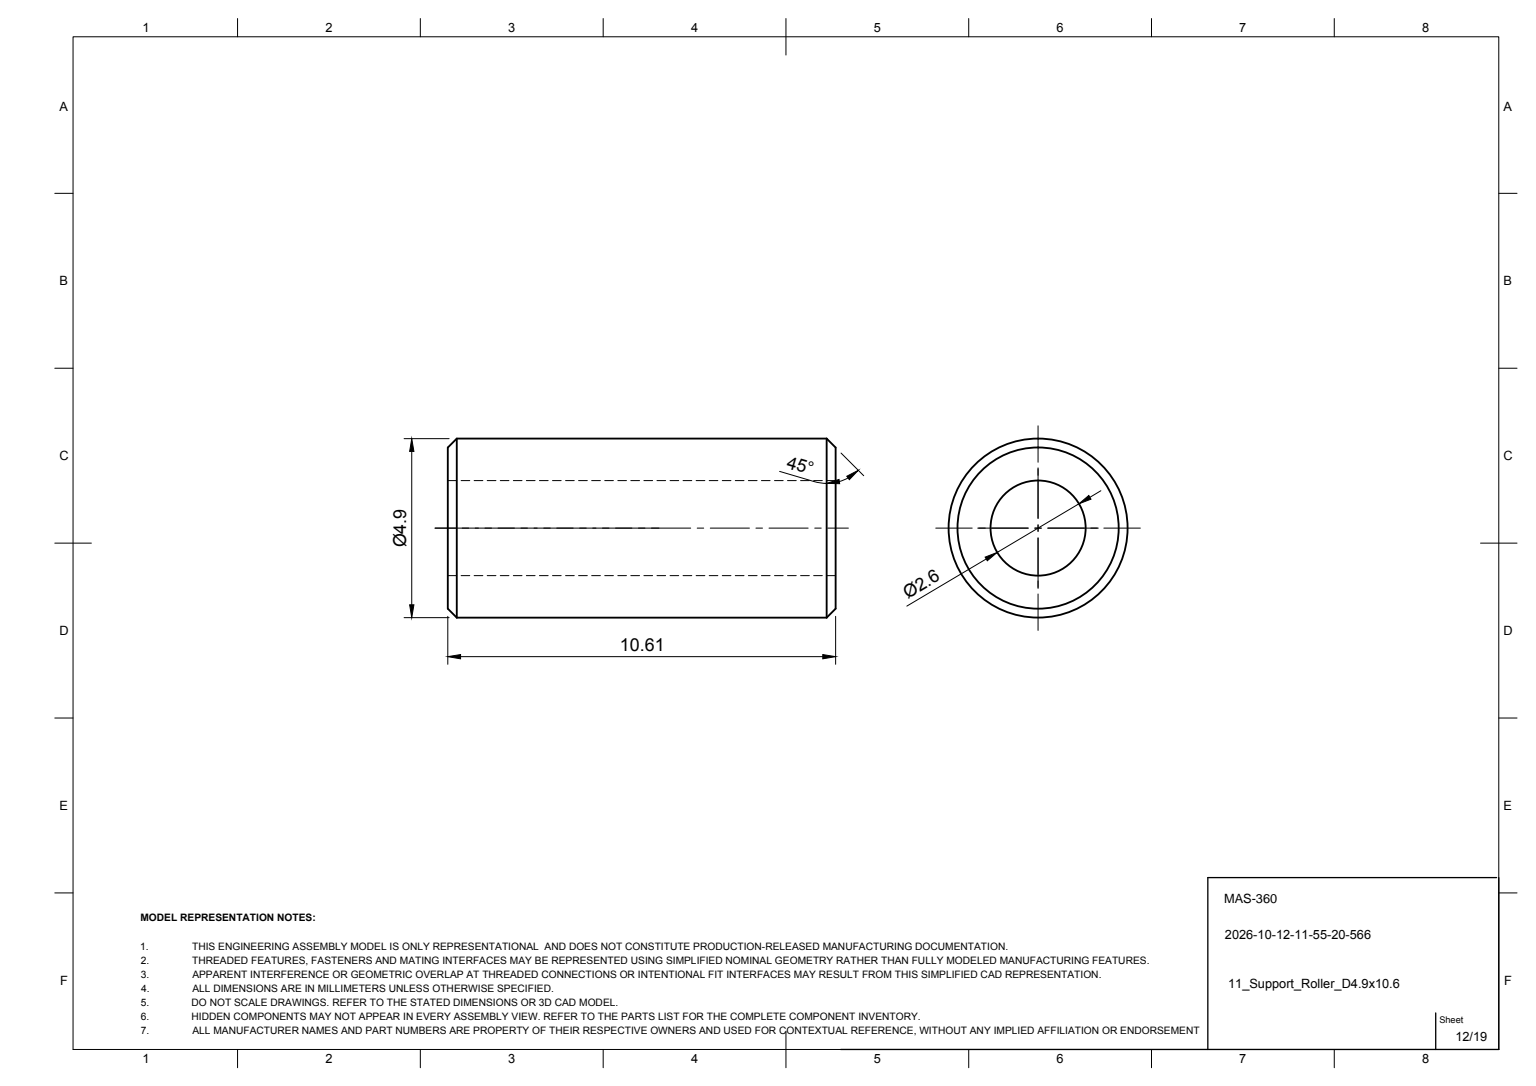
ISO-10303-21;
HEADER;
/* Generated by software containing ST-Developer
 * from STEP Tools, Inc. (www.steptools.com) 
 */

FILE_DESCRIPTION(
/* description */ (''),
/* implementation_level */ '2;1');

FILE_NAME(
/* name */ '11_Support_Roller_D4.9x10.6.step',
/* time_stamp */ '2026-11-04T18:53:29-08:00',
/* author */ (''),
/* organization */ (''),
/* preprocessor_version */ 'ST-DEVELOPER v20.2',
/* originating_system */ 'Autodesk Translation Framework v15.17.0.0',
/* authorisation */ '');

FILE_SCHEMA (('AUTOMOTIVE_DESIGN { 1 0 10303 214 3 1 1 }'));
ENDSEC;

DATA;
#10=MECHANICAL_DESIGN_GEOMETRIC_PRESENTATION_REPRESENTATION('',(#1338),#100031);
#237=CONICAL_SURFACE('',#22405,2.3256,0.785398163397447);
#238=CONICAL_SURFACE('',#22410,2.3256,0.785398163397447);
#1142=CIRCLE('',#22406,2.448);
#1143=CIRCLE('',#22407,2.2032);
#1144=CIRCLE('',#22409,2.448);
#1145=CIRCLE('',#22411,2.2032);
#1146=CIRCLE('',#22413,1.3);
#1147=CIRCLE('',#22415,1.3);
#1302=SHAPE_REPRESENTATION_RELATIONSHIP('SRR','None',#100112,#1320);
#1320=ADVANCED_BREP_SHAPE_REPRESENTATION('',(#1356),#100024);
#1338=STYLED_ITEM('',(#100200),#1356);
#1356=MANIFOLD_SOLID_BREP('Body1',#20128);
#1675=PLANE('',#22412);
#1676=PLANE('',#22416);
#1802=FACE_BOUND('',#7405,.T.);
#1803=FACE_BOUND('',#7408,.T.);
#3241=LINE('',#99809,#4528);
#3242=LINE('',#99814,#4529);
#3243=LINE('',#99817,#4530);
#3244=LINE('',#99825,#4531);
#4528=VECTOR('',#27932,2.3256);
#4529=VECTOR('',#27939,2.448);
#4530=VECTOR('',#27942,2.3256);
#4531=VECTOR('',#27953,1.3);
#5013=CYLINDRICAL_SURFACE('',#22408,2.448);
#5014=CYLINDRICAL_SURFACE('',#22414,1.3);
#6136=FACE_OUTER_BOUND('',#7401,.T.);
#6137=FACE_OUTER_BOUND('',#7402,.T.);
#6138=FACE_OUTER_BOUND('',#7403,.T.);
#6139=FACE_OUTER_BOUND('',#7404,.T.);
#6140=FACE_OUTER_BOUND('',#7406,.T.);
#6141=FACE_OUTER_BOUND('',#7407,.T.);
#7401=EDGE_LOOP('',(#18715,#18716,#18717,#18718));
#7402=EDGE_LOOP('',(#18719,#18720,#18721,#18722));
#7403=EDGE_LOOP('',(#18723,#18724,#18725,#18726));
#7404=EDGE_LOOP('',(#18727));
#7405=EDGE_LOOP('',(#18728));
#7406=EDGE_LOOP('',(#18729,#18730,#18731,#18732));
#7407=EDGE_LOOP('',(#18733));
#7408=EDGE_LOOP('',(#18734));
#9883=VERTEX_POINT('',#99806);
#9884=VERTEX_POINT('',#99808);
#9885=VERTEX_POINT('',#99812);
#9886=VERTEX_POINT('',#99816);
#9887=VERTEX_POINT('',#99820);
#9888=VERTEX_POINT('',#99823);
#12832=EDGE_CURVE('',#9883,#9883,#1142,.T.);
#12833=EDGE_CURVE('',#9883,#9884,#3241,.T.);
#12834=EDGE_CURVE('',#9884,#9884,#1143,.T.);
#12835=EDGE_CURVE('',#9885,#9885,#1144,.T.);
#12836=EDGE_CURVE('',#9885,#9883,#3242,.T.);
#12837=EDGE_CURVE('',#9885,#9886,#3243,.T.);
#12838=EDGE_CURVE('',#9886,#9886,#1145,.T.);
#12839=EDGE_CURVE('',#9887,#9887,#1146,.T.);
#12840=EDGE_CURVE('',#9888,#9888,#1147,.T.);
#12841=EDGE_CURVE('',#9888,#9887,#3244,.T.);
#18715=ORIENTED_EDGE('',*,*,#12832,.F.);
#18716=ORIENTED_EDGE('',*,*,#12833,.T.);
#18717=ORIENTED_EDGE('',*,*,#12834,.T.);
#18718=ORIENTED_EDGE('',*,*,#12833,.F.);
#18719=ORIENTED_EDGE('',*,*,#12835,.F.);
#18720=ORIENTED_EDGE('',*,*,#12836,.T.);
#18721=ORIENTED_EDGE('',*,*,#12832,.T.);
#18722=ORIENTED_EDGE('',*,*,#12836,.F.);
#18723=ORIENTED_EDGE('',*,*,#12835,.T.);
#18724=ORIENTED_EDGE('',*,*,#12837,.T.);
#18725=ORIENTED_EDGE('',*,*,#12838,.F.);
#18726=ORIENTED_EDGE('',*,*,#12837,.F.);
#18727=ORIENTED_EDGE('',*,*,#12838,.T.);
#18728=ORIENTED_EDGE('',*,*,#12839,.F.);
#18729=ORIENTED_EDGE('',*,*,#12840,.F.);
#18730=ORIENTED_EDGE('',*,*,#12841,.T.);
#18731=ORIENTED_EDGE('',*,*,#12839,.T.);
#18732=ORIENTED_EDGE('',*,*,#12841,.F.);
#18733=ORIENTED_EDGE('',*,*,#12834,.F.);
#18734=ORIENTED_EDGE('',*,*,#12840,.T.);
#20070=ADVANCED_FACE('',(#6136),#237,.T.);
#20071=ADVANCED_FACE('',(#6137),#5013,.T.);
#20072=ADVANCED_FACE('',(#6138),#238,.T.);
#20073=ADVANCED_FACE('',(#6139,#1802),#1675,.T.);
#20074=ADVANCED_FACE('',(#6140),#5014,.F.);
#20075=ADVANCED_FACE('',(#6141,#1803),#1676,.T.);
#20128=CLOSED_SHELL('',(#20070,#20071,#20072,#20073,#20074,#20075));
#22404=AXIS2_PLACEMENT_3D('',#99804,#27926,#27927);
#22405=AXIS2_PLACEMENT_3D('',#99805,#27928,#27929);
#22406=AXIS2_PLACEMENT_3D('',#99807,#27930,#27931);
#22407=AXIS2_PLACEMENT_3D('',#99810,#27933,#27934);
#22408=AXIS2_PLACEMENT_3D('',#99811,#27935,#27936);
#22409=AXIS2_PLACEMENT_3D('',#99813,#27937,#27938);
#22410=AXIS2_PLACEMENT_3D('',#99815,#27940,#27941);
#22411=AXIS2_PLACEMENT_3D('',#99818,#27943,#27944);
#22412=AXIS2_PLACEMENT_3D('',#99819,#27945,#27946);
#22413=AXIS2_PLACEMENT_3D('',#99821,#27947,#27948);
#22414=AXIS2_PLACEMENT_3D('',#99822,#27949,#27950);
#22415=AXIS2_PLACEMENT_3D('',#99824,#27951,#27952);
#22416=AXIS2_PLACEMENT_3D('',#99826,#27954,#27955);
#27926=DIRECTION('axis',(0.,0.,1.));
#27927=DIRECTION('refdir',(1.,0.,0.));
#27928=DIRECTION('center_axis',(1.,0.,0.));
#27929=DIRECTION('ref_axis',(0.,1.,0.));
#27930=DIRECTION('center_axis',(1.,0.,0.));
#27931=DIRECTION('ref_axis',(0.,0.,-1.));
#27932=DIRECTION('',(-0.707106781186548,0.707106781186547,8.65956056235492E-17));
#27933=DIRECTION('center_axis',(1.,0.,0.));
#27934=DIRECTION('ref_axis',(0.,0.,-1.));
#27935=DIRECTION('center_axis',(1.,0.,0.));
#27936=DIRECTION('ref_axis',(0.,1.,0.));
#27937=DIRECTION('center_axis',(1.,0.,0.));
#27938=DIRECTION('ref_axis',(0.,0.,-1.));
#27939=DIRECTION('',(-1.,0.,0.));
#27940=DIRECTION('center_axis',(-1.,0.,0.));
#27941=DIRECTION('ref_axis',(0.,1.,0.));
#27942=DIRECTION('',(0.707106781186548,0.707106781186547,-8.65956056235492E-17));
#27943=DIRECTION('center_axis',(1.,0.,0.));
#27944=DIRECTION('ref_axis',(0.,0.,-1.));
#27945=DIRECTION('center_axis',(1.,0.,0.));
#27946=DIRECTION('ref_axis',(0.,0.,-1.));
#27947=DIRECTION('center_axis',(1.,0.,0.));
#27948=DIRECTION('ref_axis',(0.,0.,-1.));
#27949=DIRECTION('center_axis',(1.,0.,0.));
#27950=DIRECTION('ref_axis',(0.,1.,0.));
#27951=DIRECTION('center_axis',(1.,0.,0.));
#27952=DIRECTION('ref_axis',(0.,0.,-1.));
#27953=DIRECTION('',(1.,0.,0.));
#27954=DIRECTION('center_axis',(-1.,0.,0.));
#27955=DIRECTION('ref_axis',(0.,0.,1.));
#99804=CARTESIAN_POINT('',(0.,0.,0.));
#99805=CARTESIAN_POINT('Origin',(-5.1816,0.,0.));
#99806=CARTESIAN_POINT('',(-5.0592,-2.448,-2.99793536431272E-16));
#99807=CARTESIAN_POINT('Origin',(-5.0592,0.,0.));
#99808=CARTESIAN_POINT('',(-5.304,-2.2032,-2.69814182788145E-16));
#99809=CARTESIAN_POINT('',(-5.1816,-2.3256,-2.84803859609709E-16));
#99810=CARTESIAN_POINT('Origin',(-5.304,0.,0.));
#99811=CARTESIAN_POINT('Origin',(0.,0.,0.));
#99812=CARTESIAN_POINT('',(5.0592,-2.448,-2.99793536431272E-16));
#99813=CARTESIAN_POINT('Origin',(5.0592,0.,0.));
#99814=CARTESIAN_POINT('',(0.,-2.448,-2.99793536431272E-16));
#99815=CARTESIAN_POINT('Origin',(5.1816,0.,0.));
#99816=CARTESIAN_POINT('',(5.304,-2.2032,-2.69814182788145E-16));
#99817=CARTESIAN_POINT('',(5.1816,-2.3256,2.84803859609709E-16));
#99818=CARTESIAN_POINT('Origin',(5.304,0.,0.));
#99819=CARTESIAN_POINT('Origin',(5.304,1.3,0.));
#99820=CARTESIAN_POINT('',(5.304,-1.3,-1.59204083889156E-16));
#99821=CARTESIAN_POINT('Origin',(5.304,0.,0.));
#99822=CARTESIAN_POINT('Origin',(0.,0.,0.));
#99823=CARTESIAN_POINT('',(-5.304,-1.3,-1.59204083889156E-16));
#99824=CARTESIAN_POINT('Origin',(-5.304,0.,0.));
#99825=CARTESIAN_POINT('',(0.,-1.3,-1.59204083889156E-16));
#99826=CARTESIAN_POINT('Origin',(-5.304,2.2032,0.));
#100004=UNCERTAINTY_MEASURE_WITH_UNIT(LENGTH_MEASURE(0.01),#100032,
'DISTANCE_ACCURACY_VALUE',
'Maximum model space distance between geometric entities at asserted c
onnectivities');
#100011=UNCERTAINTY_MEASURE_WITH_UNIT(LENGTH_MEASURE(0.01),#100032,
'DISTANCE_ACCURACY_VALUE',
'Maximum model space distance between geometric entities at asserted c
onnectivities');
#100024=(
GEOMETRIC_REPRESENTATION_CONTEXT(3)
GLOBAL_UNCERTAINTY_ASSIGNED_CONTEXT((#100004))
GLOBAL_UNIT_ASSIGNED_CONTEXT((#100032,#100034,#100035))
REPRESENTATION_CONTEXT('','3D')
);
#100031=(
GEOMETRIC_REPRESENTATION_CONTEXT(3)
GLOBAL_UNCERTAINTY_ASSIGNED_CONTEXT((#100011))
GLOBAL_UNIT_ASSIGNED_CONTEXT((#100032,#100034,#100035))
REPRESENTATION_CONTEXT('','3D')
);
#100032=(
LENGTH_UNIT()
NAMED_UNIT(*)
SI_UNIT(.MILLI.,.METRE.)
);
#100034=(
NAMED_UNIT(*)
PLANE_ANGLE_UNIT()
SI_UNIT($,.RADIAN.)
);
#100035=(
NAMED_UNIT(*)
SI_UNIT($,.STERADIAN.)
SOLID_ANGLE_UNIT()
);
#100048=SHAPE_DEFINITION_REPRESENTATION(#100067,#100112);
#100067=PRODUCT_DEFINITION_SHAPE('',$,#100132);
#100112=SHAPE_REPRESENTATION('',(#22404),#100024);
#100119=PRODUCT_DEFINITION_CONTEXT('part definition',#100178,'design');
#100132=PRODUCT_DEFINITION('2026-10-12-11-55-20-566',
'11_Support_Roller_D4.9x10.6',#100151,#100119);
#100151=PRODUCT_DEFINITION_FORMATION('',$,#100192);
#100178=APPLICATION_CONTEXT(
'Core Data for Automotive Mechanical Design Process');
#100179=PRODUCT_CONTEXT('part definition',#100178,'mechanical');
#100192=PRODUCT('2026-10-12-11-55-20-566','11_Support_Roller_D4.9x10.6',
$,(#100179));
#100200=PRESENTATION_STYLE_ASSIGNMENT((#100206));
#100206=SURFACE_STYLE_USAGE(.BOTH.,#100212);
#100212=SURFACE_SIDE_STYLE('',(#100218));
#100218=SURFACE_STYLE_FILL_AREA(#100224);
#100224=FILL_AREA_STYLE('Opaque(227,224,212)',(#100230));
#100230=FILL_AREA_STYLE_COLOUR('Opaque(227,224,212)',#100236);
#100236=COLOUR_RGB('Opaque(227,224,212)',0.890196078431372,0.87843137254902,
0.831372549019608);
ENDSEC;
END-ISO-10303-21;
